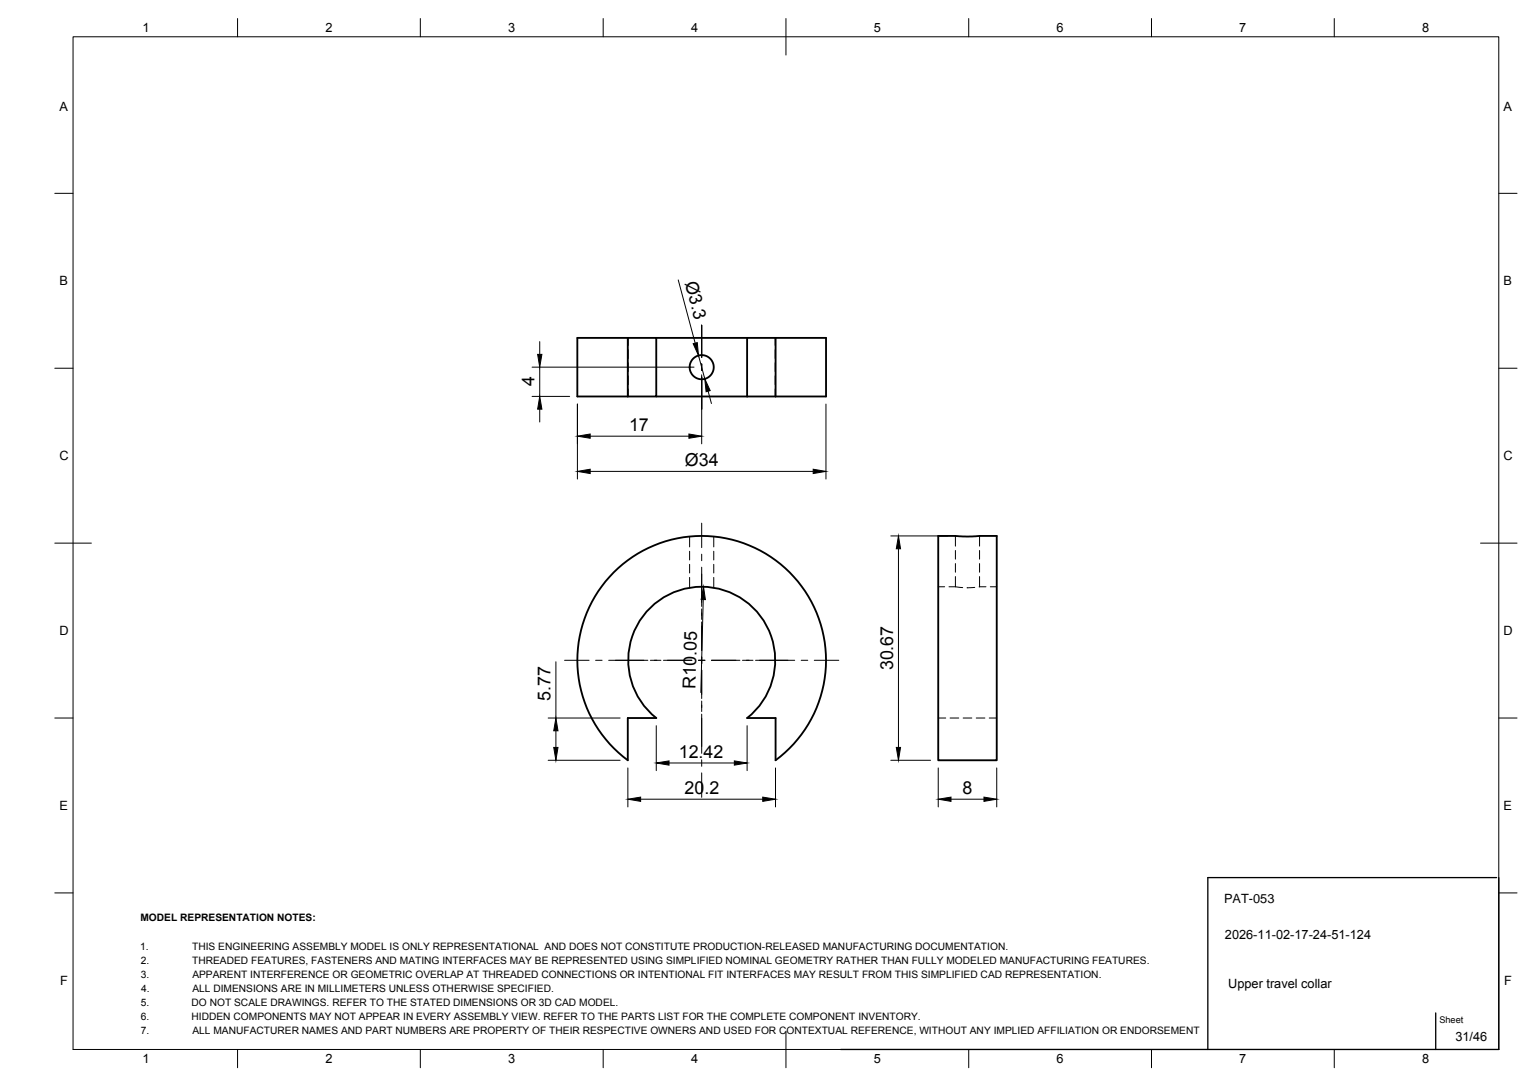
ISO-10303-21;
HEADER;
/* Generated by software containing ST-Developer
 * from STEP Tools, Inc. (www.steptools.com) 
 */

FILE_DESCRIPTION(
/* description */ ('Hand-operated arbor press'),
/* implementation_level */ '2;1');

FILE_NAME(
/* name */ 'Upper travel collar.step',
/* time_stamp */ '2026-10-28T03:25:25-07:00',
/* author */ (''),
/* organization */ (''),
/* preprocessor_version */ 'ST-DEVELOPER v20.2',
/* originating_system */ 'Autodesk Translation Framework v15.17.0.0',
/* authorisation */ '');

FILE_SCHEMA (('AUTOMOTIVE_DESIGN { 1 0 10303 214 3 1 1 }'));
ENDSEC;

DATA;
#10=MECHANICAL_DESIGN_GEOMETRIC_PRESENTATION_REPRESENTATION('',(#617),#32751);
#453=B_SPLINE_CURVE_WITH_KNOTS('',3,(#20353,#20354,#20355,#20356,#20357,
#20358,#20359,#20360,#20361,#20362),.UNSPECIFIED.,.F.,.F.,(4,2,2,2,4),(0.,
0.0622753849594643,0.124550769918929,0.186824589898795,0.249098409878661),
 .UNSPECIFIED.);
#454=B_SPLINE_CURVE_WITH_KNOTS('',3,(#20363,#20364,#20365,#20366,#20367,
#20368,#20369,#20370,#20371,#20372,#20373,#20374,#20375,#20376,#20377,#20378,
#20379,#20380,#20381,#20382,#20383,#20384,#20385,#20386,#20387,#20388),
 .UNSPECIFIED.,.F.,.F.,(4,2,2,2,2,2,2,2,2,2,2,2,4),(0.249098409878661,0.311372229858528,
0.373646049838394,0.435921434797858,0.498196819757323,0.560472204716787,
0.622747589676251,0.685021409656117,0.747295229635984,0.80956904961585,
0.871842869595717,0.934118254555181,0.996393639514645),.UNSPECIFIED.);
#455=B_SPLINE_CURVE_WITH_KNOTS('',3,(#20392,#20393,#20394,#20395,#20396,
#20397,#20398,#20399,#20400,#20401,#20402,#20403,#20404,#20405,#20406,#20407,
#20408,#20409,#20410,#20411,#20412,#20413,#20414,#20415,#20416,#20417),
 .UNSPECIFIED.,.F.,.F.,(4,2,2,2,2,2,2,2,2,2,2,2,4),(0.,0.0621954302022346,
0.124390860404469,0.186586102839082,0.248781345273694,0.310976587708307,
0.37317183014292,0.435367260345154,0.497562690547389,0.559758120749623,
0.621953550951858,0.68414879338647,0.746344035821083),.UNSPECIFIED.);
#456=B_SPLINE_CURVE_WITH_KNOTS('',3,(#20418,#20419,#20420,#20421,#20422,
#20423,#20424,#20425,#20426,#20427),.UNSPECIFIED.,.F.,.F.,(4,2,2,2,4),(0.746344035821083,
0.808539278255696,0.870734520690308,0.932929950892543,0.995125381094778),
 .UNSPECIFIED.);
#526=SHAPE_REPRESENTATION_RELATIONSHIP('SRR','None',#32957,#568);
#568=ADVANCED_BREP_SHAPE_REPRESENTATION('',(#664),#32731);
#617=STYLED_ITEM('',(#33228),#664);
#664=MANIFOLD_SOLID_BREP('Body1',#12516);
#814=FACE_BOUND('',#2575,.T.);
#815=FACE_BOUND('',#2577,.T.);
#1177=PLANE('',#13760);
#1178=PLANE('',#13761);
#1179=PLANE('',#13762);
#1180=PLANE('',#13763);
#1181=PLANE('',#13764);
#1182=PLANE('',#13771);
#1753=FACE_OUTER_BOUND('',#2568,.T.);
#1754=FACE_OUTER_BOUND('',#2569,.T.);
#1755=FACE_OUTER_BOUND('',#2570,.T.);
#1756=FACE_OUTER_BOUND('',#2571,.T.);
#1757=FACE_OUTER_BOUND('',#2572,.T.);
#1758=FACE_OUTER_BOUND('',#2573,.T.);
#1759=FACE_OUTER_BOUND('',#2574,.T.);
#1760=FACE_OUTER_BOUND('',#2576,.T.);
#1761=FACE_OUTER_BOUND('',#2578,.T.);
#2568=EDGE_LOOP('',(#10626,#10627,#10628,#10629,#10630,#10631));
#2569=EDGE_LOOP('',(#10632,#10633,#10634,#10635));
#2570=EDGE_LOOP('',(#10636,#10637,#10638,#10639));
#2571=EDGE_LOOP('',(#10640,#10641,#10642,#10643));
#2572=EDGE_LOOP('',(#10644,#10645,#10646,#10647));
#2573=EDGE_LOOP('',(#10648,#10649,#10650,#10651,#10652,#10653));
#2574=EDGE_LOOP('',(#10654,#10655,#10656,#10657));
#2575=EDGE_LOOP('',(#10658,#10659));
#2576=EDGE_LOOP('',(#10660,#10661,#10662,#10663));
#2577=EDGE_LOOP('',(#10664,#10665));
#2578=EDGE_LOOP('',(#10666,#10667,#10668,#10669,#10670,#10671));
#3695=LINE('',#20390,#4866);
#3696=LINE('',#20431,#4867);
#3697=LINE('',#20433,#4868);
#3698=LINE('',#20435,#4869);
#3699=LINE('',#20436,#4870);
#3700=LINE('',#20440,#4871);
#3701=LINE('',#20442,#4872);
#3702=LINE('',#20444,#4873);
#3703=LINE('',#20445,#4874);
#3704=LINE('',#20448,#4875);
#3705=LINE('',#20450,#4876);
#3706=LINE('',#20451,#4877);
#3707=LINE('',#20454,#4878);
#3708=LINE('',#20456,#4879);
#3709=LINE('',#20457,#4880);
#4866=VECTOR('',#16548,0.164999999999999);
#4867=VECTOR('',#16551,1.);
#4868=VECTOR('',#16552,1.);
#4869=VECTOR('',#16553,1.);
#4870=VECTOR('',#16554,1.);
#4871=VECTOR('',#16557,1.);
#4872=VECTOR('',#16558,1.);
#4873=VECTOR('',#16559,1.);
#4874=VECTOR('',#16560,1.);
#4875=VECTOR('',#16563,1.);
#4876=VECTOR('',#16564,1.);
#4877=VECTOR('',#16565,1.);
#4878=VECTOR('',#16568,1.);
#4879=VECTOR('',#16569,1.);
#4880=VECTOR('',#16570,1.);
#5432=CIRCLE('',#13765,1.005);
#5433=CIRCLE('',#13766,1.7);
#5434=CIRCLE('',#13768,1.7);
#5435=CIRCLE('',#13770,1.005);
#6329=VERTEX_POINT('',#20351);
#6330=VERTEX_POINT('',#20352);
#6331=VERTEX_POINT('',#20389);
#6332=VERTEX_POINT('',#20391);
#6333=VERTEX_POINT('',#20429);
#6334=VERTEX_POINT('',#20430);
#6335=VERTEX_POINT('',#20432);
#6336=VERTEX_POINT('',#20434);
#6337=VERTEX_POINT('',#20438);
#6338=VERTEX_POINT('',#20439);
#6339=VERTEX_POINT('',#20441);
#6340=VERTEX_POINT('',#20443);
#6341=VERTEX_POINT('',#20447);
#6342=VERTEX_POINT('',#20449);
#6343=VERTEX_POINT('',#20453);
#6344=VERTEX_POINT('',#20455);
#7816=EDGE_CURVE('',#6329,#6330,#453,.T.);
#7817=EDGE_CURVE('',#6330,#6329,#454,.T.);
#7818=EDGE_CURVE('',#6330,#6331,#3695,.T.);
#7819=EDGE_CURVE('',#6332,#6331,#455,.T.);
#7820=EDGE_CURVE('',#6331,#6332,#456,.T.);
#7821=EDGE_CURVE('',#6333,#6334,#3696,.T.);
#7822=EDGE_CURVE('',#6333,#6335,#3697,.T.);
#7823=EDGE_CURVE('',#6336,#6335,#3698,.T.);
#7824=EDGE_CURVE('',#6334,#6336,#3699,.T.);
#7825=EDGE_CURVE('',#6337,#6338,#3700,.T.);
#7826=EDGE_CURVE('',#6337,#6339,#3701,.T.);
#7827=EDGE_CURVE('',#6340,#6339,#3702,.T.);
#7828=EDGE_CURVE('',#6338,#6340,#3703,.T.);
#7829=EDGE_CURVE('',#6341,#6333,#3704,.T.);
#7830=EDGE_CURVE('',#6342,#6341,#3705,.T.);
#7831=EDGE_CURVE('',#6335,#6342,#3706,.T.);
#7832=EDGE_CURVE('',#6343,#6337,#3707,.T.);
#7833=EDGE_CURVE('',#6344,#6343,#3708,.T.);
#7834=EDGE_CURVE('',#6339,#6344,#3709,.T.);
#7835=EDGE_CURVE('',#6342,#6340,#5432,.T.);
#7836=EDGE_CURVE('',#6344,#6336,#5433,.T.);
#7837=EDGE_CURVE('',#6343,#6334,#5434,.T.);
#7838=EDGE_CURVE('',#6341,#6338,#5435,.T.);
#10626=ORIENTED_EDGE('',*,*,#7816,.F.);
#10627=ORIENTED_EDGE('',*,*,#7817,.F.);
#10628=ORIENTED_EDGE('',*,*,#7818,.T.);
#10629=ORIENTED_EDGE('',*,*,#7819,.F.);
#10630=ORIENTED_EDGE('',*,*,#7820,.F.);
#10631=ORIENTED_EDGE('',*,*,#7818,.F.);
#10632=ORIENTED_EDGE('',*,*,#7821,.F.);
#10633=ORIENTED_EDGE('',*,*,#7822,.T.);
#10634=ORIENTED_EDGE('',*,*,#7823,.F.);
#10635=ORIENTED_EDGE('',*,*,#7824,.F.);
#10636=ORIENTED_EDGE('',*,*,#7825,.F.);
#10637=ORIENTED_EDGE('',*,*,#7826,.T.);
#10638=ORIENTED_EDGE('',*,*,#7827,.F.);
#10639=ORIENTED_EDGE('',*,*,#7828,.F.);
#10640=ORIENTED_EDGE('',*,*,#7829,.F.);
#10641=ORIENTED_EDGE('',*,*,#7830,.F.);
#10642=ORIENTED_EDGE('',*,*,#7831,.F.);
#10643=ORIENTED_EDGE('',*,*,#7822,.F.);
#10644=ORIENTED_EDGE('',*,*,#7832,.F.);
#10645=ORIENTED_EDGE('',*,*,#7833,.F.);
#10646=ORIENTED_EDGE('',*,*,#7834,.F.);
#10647=ORIENTED_EDGE('',*,*,#7826,.F.);
#10648=ORIENTED_EDGE('',*,*,#7823,.T.);
#10649=ORIENTED_EDGE('',*,*,#7831,.T.);
#10650=ORIENTED_EDGE('',*,*,#7835,.T.);
#10651=ORIENTED_EDGE('',*,*,#7827,.T.);
#10652=ORIENTED_EDGE('',*,*,#7834,.T.);
#10653=ORIENTED_EDGE('',*,*,#7836,.T.);
#10654=ORIENTED_EDGE('',*,*,#7824,.T.);
#10655=ORIENTED_EDGE('',*,*,#7836,.F.);
#10656=ORIENTED_EDGE('',*,*,#7833,.T.);
#10657=ORIENTED_EDGE('',*,*,#7837,.T.);
#10658=ORIENTED_EDGE('',*,*,#7819,.T.);
#10659=ORIENTED_EDGE('',*,*,#7820,.T.);
#10660=ORIENTED_EDGE('',*,*,#7830,.T.);
#10661=ORIENTED_EDGE('',*,*,#7838,.T.);
#10662=ORIENTED_EDGE('',*,*,#7828,.T.);
#10663=ORIENTED_EDGE('',*,*,#7835,.F.);
#10664=ORIENTED_EDGE('',*,*,#7816,.T.);
#10665=ORIENTED_EDGE('',*,*,#7817,.T.);
#10666=ORIENTED_EDGE('',*,*,#7821,.T.);
#10667=ORIENTED_EDGE('',*,*,#7837,.F.);
#10668=ORIENTED_EDGE('',*,*,#7832,.T.);
#10669=ORIENTED_EDGE('',*,*,#7825,.T.);
#10670=ORIENTED_EDGE('',*,*,#7838,.F.);
#10671=ORIENTED_EDGE('',*,*,#7829,.T.);
#11747=CYLINDRICAL_SURFACE('',#13759,0.164999999999999);
#11748=CYLINDRICAL_SURFACE('',#13767,1.7);
#11749=CYLINDRICAL_SURFACE('',#13769,1.005);
#12262=ADVANCED_FACE('',(#1753),#11747,.F.);
#12263=ADVANCED_FACE('',(#1754),#1177,.F.);
#12264=ADVANCED_FACE('',(#1755),#1178,.F.);
#12265=ADVANCED_FACE('',(#1756),#1179,.F.);
#12266=ADVANCED_FACE('',(#1757),#1180,.F.);
#12267=ADVANCED_FACE('',(#1758),#1181,.T.);
#12268=ADVANCED_FACE('',(#1759,#814),#11748,.T.);
#12269=ADVANCED_FACE('',(#1760,#815),#11749,.F.);
#12270=ADVANCED_FACE('',(#1761),#1182,.F.);
#12516=CLOSED_SHELL('',(#12262,#12263,#12264,#12265,#12266,#12267,#12268,
#12269,#12270));
#13758=AXIS2_PLACEMENT_3D('',#20349,#16544,#16545);
#13759=AXIS2_PLACEMENT_3D('',#20350,#16546,#16547);
#13760=AXIS2_PLACEMENT_3D('',#20428,#16549,#16550);
#13761=AXIS2_PLACEMENT_3D('',#20437,#16555,#16556);
#13762=AXIS2_PLACEMENT_3D('',#20446,#16561,#16562);
#13763=AXIS2_PLACEMENT_3D('',#20452,#16566,#16567);
#13764=AXIS2_PLACEMENT_3D('',#20458,#16571,#16572);
#13765=AXIS2_PLACEMENT_3D('',#20459,#16573,#16574);
#13766=AXIS2_PLACEMENT_3D('',#20460,#16575,#16576);
#13767=AXIS2_PLACEMENT_3D('',#20461,#16577,#16578);
#13768=AXIS2_PLACEMENT_3D('',#20462,#16579,#16580);
#13769=AXIS2_PLACEMENT_3D('',#20463,#16581,#16582);
#13770=AXIS2_PLACEMENT_3D('',#20464,#16583,#16584);
#13771=AXIS2_PLACEMENT_3D('',#20465,#16585,#16586);
#16544=DIRECTION('axis',(0.,0.,1.));
#16545=DIRECTION('refdir',(1.,0.,0.));
#16546=DIRECTION('center_axis',(1.,0.,0.));
#16547=DIRECTION('ref_axis',(0.,0.,-1.));
#16548=DIRECTION('',(1.,0.,0.));
#16549=DIRECTION('center_axis',(0.,1.,0.));
#16550=DIRECTION('ref_axis',(-1.,0.,0.));
#16551=DIRECTION('',(-1.,0.,0.));
#16552=DIRECTION('',(0.,0.,1.));
#16553=DIRECTION('',(1.,0.,0.));
#16554=DIRECTION('',(0.,0.,1.));
#16555=DIRECTION('center_axis',(1.,0.,0.));
#16556=DIRECTION('ref_axis',(0.,1.,0.));
#16557=DIRECTION('',(0.,1.,0.));
#16558=DIRECTION('',(0.,0.,1.));
#16559=DIRECTION('',(0.,-1.,0.));
#16560=DIRECTION('',(0.,0.,1.));
#16561=DIRECTION('center_axis',(1.,0.,0.));
#16562=DIRECTION('ref_axis',(0.,1.,0.));
#16563=DIRECTION('',(0.,1.,0.));
#16564=DIRECTION('',(0.,0.,-1.));
#16565=DIRECTION('',(0.,-1.,0.));
#16566=DIRECTION('center_axis',(0.,-1.,0.));
#16567=DIRECTION('ref_axis',(1.,0.,0.));
#16568=DIRECTION('',(1.,0.,0.));
#16569=DIRECTION('',(0.,0.,-1.));
#16570=DIRECTION('',(-1.,0.,0.));
#16571=DIRECTION('center_axis',(0.,0.,1.));
#16572=DIRECTION('ref_axis',(1.,0.,0.));
#16573=DIRECTION('center_axis',(0.,0.,-1.));
#16574=DIRECTION('ref_axis',(1.,0.,0.));
#16575=DIRECTION('center_axis',(0.,0.,1.));
#16576=DIRECTION('ref_axis',(1.,0.,0.));
#16577=DIRECTION('center_axis',(0.,0.,1.));
#16578=DIRECTION('ref_axis',(1.,0.,0.));
#16579=DIRECTION('center_axis',(0.,0.,1.));
#16580=DIRECTION('ref_axis',(1.,0.,0.));
#16581=DIRECTION('center_axis',(0.,0.,1.));
#16582=DIRECTION('ref_axis',(1.,0.,0.));
#16583=DIRECTION('center_axis',(0.,0.,-1.));
#16584=DIRECTION('ref_axis',(1.,0.,0.));
#16585=DIRECTION('center_axis',(0.,0.,1.));
#16586=DIRECTION('ref_axis',(1.,0.,0.));
#20349=CARTESIAN_POINT('',(0.,0.,0.));
#20350=CARTESIAN_POINT('Origin',(1.99,0.,34.));
#20351=CARTESIAN_POINT('',(1.9913626985115,0.164999999999999,34.));
#20352=CARTESIAN_POINT('',(2.005,3.8468921234385E-17,34.165));
#20353=CARTESIAN_POINT('Ctrl Pts',(1.9913626985115,0.164999999999999,34.));
#20354=CARTESIAN_POINT('Ctrl Pts',(1.9913626985115,0.164999999999999,34.0207584616532));
#20355=CARTESIAN_POINT('Ctrl Pts',(1.99208213234536,0.160843707720235,34.0428743626922));
#20356=CARTESIAN_POINT('Ctrl Pts',(1.99466757507705,0.143993298000807,34.0835155100945));
#20357=CARTESIAN_POINT('Ctrl Pts',(1.9964948147884,0.131301190829394,34.1020440469622));
#20358=CARTESIAN_POINT('Ctrl Pts',(1.99991441892026,0.102044414577984,34.1313008232136));
#20359=CARTESIAN_POINT('Ctrl Pts',(2.00173085232892,0.0835157197655827,
34.1439932187437));
#20360=CARTESIAN_POINT('Ctrl Pts',(2.00429148829838,0.0428740302308147,
34.1608438378879));
#20361=CARTESIAN_POINT('Ctrl Pts',(2.005,0.0207579399932883,34.165));
#20362=CARTESIAN_POINT('Ctrl Pts',(2.005,-4.78783679369599E-16,34.165));
#20363=CARTESIAN_POINT('Ctrl Pts',(2.005,9.0205620750794E-17,34.165));
#20364=CARTESIAN_POINT('Ctrl Pts',(2.005,-0.0207579399932887,34.165));
#20365=CARTESIAN_POINT('Ctrl Pts',(2.00429148829838,-0.0428740302308147,
34.1608438378879));
#20366=CARTESIAN_POINT('Ctrl Pts',(2.00173085232892,-0.0835157197655826,
34.1439932187437));
#20367=CARTESIAN_POINT('Ctrl Pts',(1.99991441892026,-0.102044414577984,
34.1313008232136));
#20368=CARTESIAN_POINT('Ctrl Pts',(1.9964948147884,-0.131301190829394,34.1020440469622));
#20369=CARTESIAN_POINT('Ctrl Pts',(1.99466757507705,-0.143993298000807,
34.0835155100945));
#20370=CARTESIAN_POINT('Ctrl Pts',(1.99208213234536,-0.160843707720235,
34.0428743626922));
#20371=CARTESIAN_POINT('Ctrl Pts',(1.9913626985115,-0.164999999999999,34.0207584616532));
#20372=CARTESIAN_POINT('Ctrl Pts',(1.9913626985115,-0.164999999999999,33.9792415383468));
#20373=CARTESIAN_POINT('Ctrl Pts',(1.99208213234536,-0.160843707720235,
33.9571256373078));
#20374=CARTESIAN_POINT('Ctrl Pts',(1.99466757507705,-0.143993298000807,
33.9164844899055));
#20375=CARTESIAN_POINT('Ctrl Pts',(1.9964948147884,-0.131301190829394,33.8979559530378));
#20376=CARTESIAN_POINT('Ctrl Pts',(1.99991441892026,-0.102044414577984,
33.8686991767864));
#20377=CARTESIAN_POINT('Ctrl Pts',(2.00173085232892,-0.0835157197655827,
33.8560067812563));
#20378=CARTESIAN_POINT('Ctrl Pts',(2.00429148829838,-0.0428740302308147,
33.8391561621121));
#20379=CARTESIAN_POINT('Ctrl Pts',(2.005,-0.0207579399932888,33.835));
#20380=CARTESIAN_POINT('Ctrl Pts',(2.005,0.0207579399932888,33.835));
#20381=CARTESIAN_POINT('Ctrl Pts',(2.00429148829838,0.0428740302308147,
33.8391561621121));
#20382=CARTESIAN_POINT('Ctrl Pts',(2.00173085232892,0.0835157197655826,
33.8560067812563));
#20383=CARTESIAN_POINT('Ctrl Pts',(1.99991441892026,0.102044414577984,33.8686991767864));
#20384=CARTESIAN_POINT('Ctrl Pts',(1.9964948147884,0.131301190829394,33.8979559530378));
#20385=CARTESIAN_POINT('Ctrl Pts',(1.99466757507705,0.143993298000807,33.9164844899055));
#20386=CARTESIAN_POINT('Ctrl Pts',(1.99208213234536,0.160843707720235,33.9571256373078));
#20387=CARTESIAN_POINT('Ctrl Pts',(1.9913626985115,0.164999999999999,33.9792415383468));
#20388=CARTESIAN_POINT('Ctrl Pts',(1.9913626985115,0.164999999999999,34.));
#20389=CARTESIAN_POINT('',(2.7,-2.02066721859312E-17,34.165));
#20390=CARTESIAN_POINT('',(1.99,-2.02066721859312E-17,34.165));
#20391=CARTESIAN_POINT('',(2.69197369955919,0.164999999999999,34.));
#20392=CARTESIAN_POINT('Ctrl Pts',(2.69197369955919,0.164999999999999,34.));
#20393=CARTESIAN_POINT('Ctrl Pts',(2.69197369955919,0.164999999999999,33.9792681899326));
#20394=CARTESIAN_POINT('Ctrl Pts',(2.69239400387291,0.160854068850875,33.9571634685398));
#20395=CARTESIAN_POINT('Ctrl Pts',(2.69391035162893,0.14401116680132,33.9165147673388));
#20396=CARTESIAN_POINT('Ctrl Pts',(2.69498430847444,0.131314908962089,33.8979696711705));
#20397=CARTESIAN_POINT('Ctrl Pts',(2.69699888419766,0.102030373034454,33.8686851352429));
#20398=CARTESIAN_POINT('Ctrl Pts',(2.69807062966546,0.0834852574625945,
33.8559888429375));
#20399=CARTESIAN_POINT('Ctrl Pts',(2.69958191522061,0.042836491374372,33.8391459150772));
#20400=CARTESIAN_POINT('Ctrl Pts',(2.7,0.0207317474782042,33.835));
#20401=CARTESIAN_POINT('Ctrl Pts',(2.7,-0.0207317474782042,33.835));
#20402=CARTESIAN_POINT('Ctrl Pts',(2.69958191522061,-0.042836491374372,
33.8391459150772));
#20403=CARTESIAN_POINT('Ctrl Pts',(2.69807062966546,-0.0834852574625945,
33.8559888429375));
#20404=CARTESIAN_POINT('Ctrl Pts',(2.69699888419766,-0.102030373034454,
33.8686851352429));
#20405=CARTESIAN_POINT('Ctrl Pts',(2.69498430847444,-0.131314908962089,
33.8979696711705));
#20406=CARTESIAN_POINT('Ctrl Pts',(2.69391035162893,-0.14401116680132,33.9165147673388));
#20407=CARTESIAN_POINT('Ctrl Pts',(2.69239400387291,-0.160854068850875,
33.9571634685398));
#20408=CARTESIAN_POINT('Ctrl Pts',(2.69197369955919,-0.164999999999999,
33.9792681899326));
#20409=CARTESIAN_POINT('Ctrl Pts',(2.69197369955919,-0.164999999999999,
34.0207318100674));
#20410=CARTESIAN_POINT('Ctrl Pts',(2.69239400387291,-0.160854068850875,
34.0428365314602));
#20411=CARTESIAN_POINT('Ctrl Pts',(2.69391035162893,-0.14401116680132,34.0834852326612));
#20412=CARTESIAN_POINT('Ctrl Pts',(2.69498430847444,-0.131314908962089,
34.1020303288295));
#20413=CARTESIAN_POINT('Ctrl Pts',(2.69699888419766,-0.102030373034454,
34.1313148647571));
#20414=CARTESIAN_POINT('Ctrl Pts',(2.69807062966546,-0.0834852574625945,
34.1440111570625));
#20415=CARTESIAN_POINT('Ctrl Pts',(2.69958191522061,-0.042836491374372,
34.1608540849228));
#20416=CARTESIAN_POINT('Ctrl Pts',(2.7,-0.0207317474782046,34.165));
#20417=CARTESIAN_POINT('Ctrl Pts',(2.7,-3.60822483003176E-16,34.165));
#20418=CARTESIAN_POINT('Ctrl Pts',(2.7,5.06539254985228E-16,34.165));
#20419=CARTESIAN_POINT('Ctrl Pts',(2.7,0.0207317474782047,34.165));
#20420=CARTESIAN_POINT('Ctrl Pts',(2.69958191522061,0.0428364913743719,
34.1608540849228));
#20421=CARTESIAN_POINT('Ctrl Pts',(2.69807062966546,0.0834852574625944,
34.1440111570625));
#20422=CARTESIAN_POINT('Ctrl Pts',(2.69699888419766,0.102030373034454,34.1313148647571));
#20423=CARTESIAN_POINT('Ctrl Pts',(2.69498430847444,0.131314908962089,34.1020303288295));
#20424=CARTESIAN_POINT('Ctrl Pts',(2.69391035162893,0.14401116680132,34.0834852326612));
#20425=CARTESIAN_POINT('Ctrl Pts',(2.69239400387291,0.160854068850875,34.0428365314602));
#20426=CARTESIAN_POINT('Ctrl Pts',(2.69197369955919,0.165,34.0207318100674));
#20427=CARTESIAN_POINT('Ctrl Pts',(2.69197369955919,0.165,34.));
#20428=CARTESIAN_POINT('Origin',(0.21,1.01,33.5));
#20429=CARTESIAN_POINT('',(0.21,1.01,33.6));
#20430=CARTESIAN_POINT('',(-0.367442869007697,1.01,33.6));
#20431=CARTESIAN_POINT('',(0.605,1.01,33.6));
#20432=CARTESIAN_POINT('',(0.21,1.01,34.4));
#20433=CARTESIAN_POINT('',(0.21,1.01,33.5));
#20434=CARTESIAN_POINT('',(-0.367442869007697,1.01,34.4));
#20435=CARTESIAN_POINT('',(0.605,1.01,34.4));
#20436=CARTESIAN_POINT('',(-0.367442869007697,1.01,33.6));
#20437=CARTESIAN_POINT('Origin',(0.21,-1.01,33.5));
#20438=CARTESIAN_POINT('',(0.21,-1.01,33.6));
#20439=CARTESIAN_POINT('',(0.21,-0.621228621362538,33.6));
#20440=CARTESIAN_POINT('',(0.21,-0.505,33.6));
#20441=CARTESIAN_POINT('',(0.21,-1.01,34.4));
#20442=CARTESIAN_POINT('',(0.21,-1.01,33.5));
#20443=CARTESIAN_POINT('',(0.21,-0.621228621362538,34.4));
#20444=CARTESIAN_POINT('',(0.21,-0.505,34.4));
#20445=CARTESIAN_POINT('',(0.21,-0.621228621362538,33.6));
#20446=CARTESIAN_POINT('Origin',(0.21,-1.01,33.5));
#20447=CARTESIAN_POINT('',(0.21,0.621228621362538,33.6));
#20448=CARTESIAN_POINT('',(0.21,-0.505,33.6));
#20449=CARTESIAN_POINT('',(0.21,0.621228621362538,34.4));
#20450=CARTESIAN_POINT('',(0.21,0.621228621362538,33.6));
#20451=CARTESIAN_POINT('',(0.21,-0.505,34.4));
#20452=CARTESIAN_POINT('Origin',(-0.8,-1.01,33.5));
#20453=CARTESIAN_POINT('',(-0.367442869007697,-1.01,33.6));
#20454=CARTESIAN_POINT('',(0.1,-1.01,33.6));
#20455=CARTESIAN_POINT('',(-0.367442869007697,-1.01,34.4));
#20456=CARTESIAN_POINT('',(-0.367442869007697,-1.01,33.6));
#20457=CARTESIAN_POINT('',(0.1,-1.01,34.4));
#20458=CARTESIAN_POINT('Origin',(1.,0.,34.4));
#20459=CARTESIAN_POINT('Origin',(1.,0.,34.4));
#20460=CARTESIAN_POINT('Origin',(1.,0.,34.4));
#20461=CARTESIAN_POINT('Origin',(1.,0.,33.6));
#20462=CARTESIAN_POINT('Origin',(1.,0.,33.6));
#20463=CARTESIAN_POINT('Origin',(1.,0.,33.6));
#20464=CARTESIAN_POINT('Origin',(1.,0.,33.6));
#20465=CARTESIAN_POINT('Origin',(1.,0.,33.6));
#32682=UNCERTAINTY_MEASURE_WITH_UNIT(LENGTH_MEASURE(0.001),#32752,
'DISTANCE_ACCURACY_VALUE',
'Maximum model space distance between geometric entities at asserted c
onnectivities');
#32702=UNCERTAINTY_MEASURE_WITH_UNIT(LENGTH_MEASURE(0.001),#32752,
'DISTANCE_ACCURACY_VALUE',
'Maximum model space distance between geometric entities at asserted c
onnectivities');
#32731=(
GEOMETRIC_REPRESENTATION_CONTEXT(3)
GLOBAL_UNCERTAINTY_ASSIGNED_CONTEXT((#32682))
GLOBAL_UNIT_ASSIGNED_CONTEXT((#32752,#32754,#32755))
REPRESENTATION_CONTEXT('','3D')
);
#32751=(
GEOMETRIC_REPRESENTATION_CONTEXT(3)
GLOBAL_UNCERTAINTY_ASSIGNED_CONTEXT((#32702))
GLOBAL_UNIT_ASSIGNED_CONTEXT((#32752,#32754,#32755))
REPRESENTATION_CONTEXT('','3D')
);
#32752=(
LENGTH_UNIT()
NAMED_UNIT(*)
SI_UNIT(.CENTI.,.METRE.)
);
#32754=(
NAMED_UNIT(*)
PLANE_ANGLE_UNIT()
SI_UNIT($,.RADIAN.)
);
#32755=(
NAMED_UNIT(*)
SI_UNIT($,.STERADIAN.)
SOLID_ANGLE_UNIT()
);
#32784=SHAPE_DEFINITION_REPRESENTATION(#32837,#32957);
#32837=PRODUCT_DEFINITION_SHAPE('',$,#33006);
#32957=SHAPE_REPRESENTATION('',(#13758),#32731);
#32977=PRODUCT_DEFINITION_CONTEXT('part definition',#33123,'design');
#33006=PRODUCT_DEFINITION('Upper travel collar','Upper travel collar',#33054,
#32977);
#33054=PRODUCT_DEFINITION_FORMATION('',$,#33153);
#33123=APPLICATION_CONTEXT(
'Core Data for Automotive Mechanical Design Process');
#33124=PRODUCT_CONTEXT('part definition',#33123,'mechanical');
#33153=PRODUCT('Upper travel collar','Upper travel collar',
'Upper travel collar',(#33124));
#33222=COLOUR_RGB('Light Blue',0.38,0.62,0.78);
#33223=FILL_AREA_STYLE_COLOUR('',#33222);
#33224=FILL_AREA_STYLE('',(#33223));
#33225=SURFACE_STYLE_FILL_AREA(#33224);
#33226=SURFACE_SIDE_STYLE('',(#33225));
#33227=SURFACE_STYLE_USAGE(.BOTH.,#33226);
#33228=PRESENTATION_STYLE_ASSIGNMENT((#33227));
ENDSEC;
END-ISO-10303-21;
